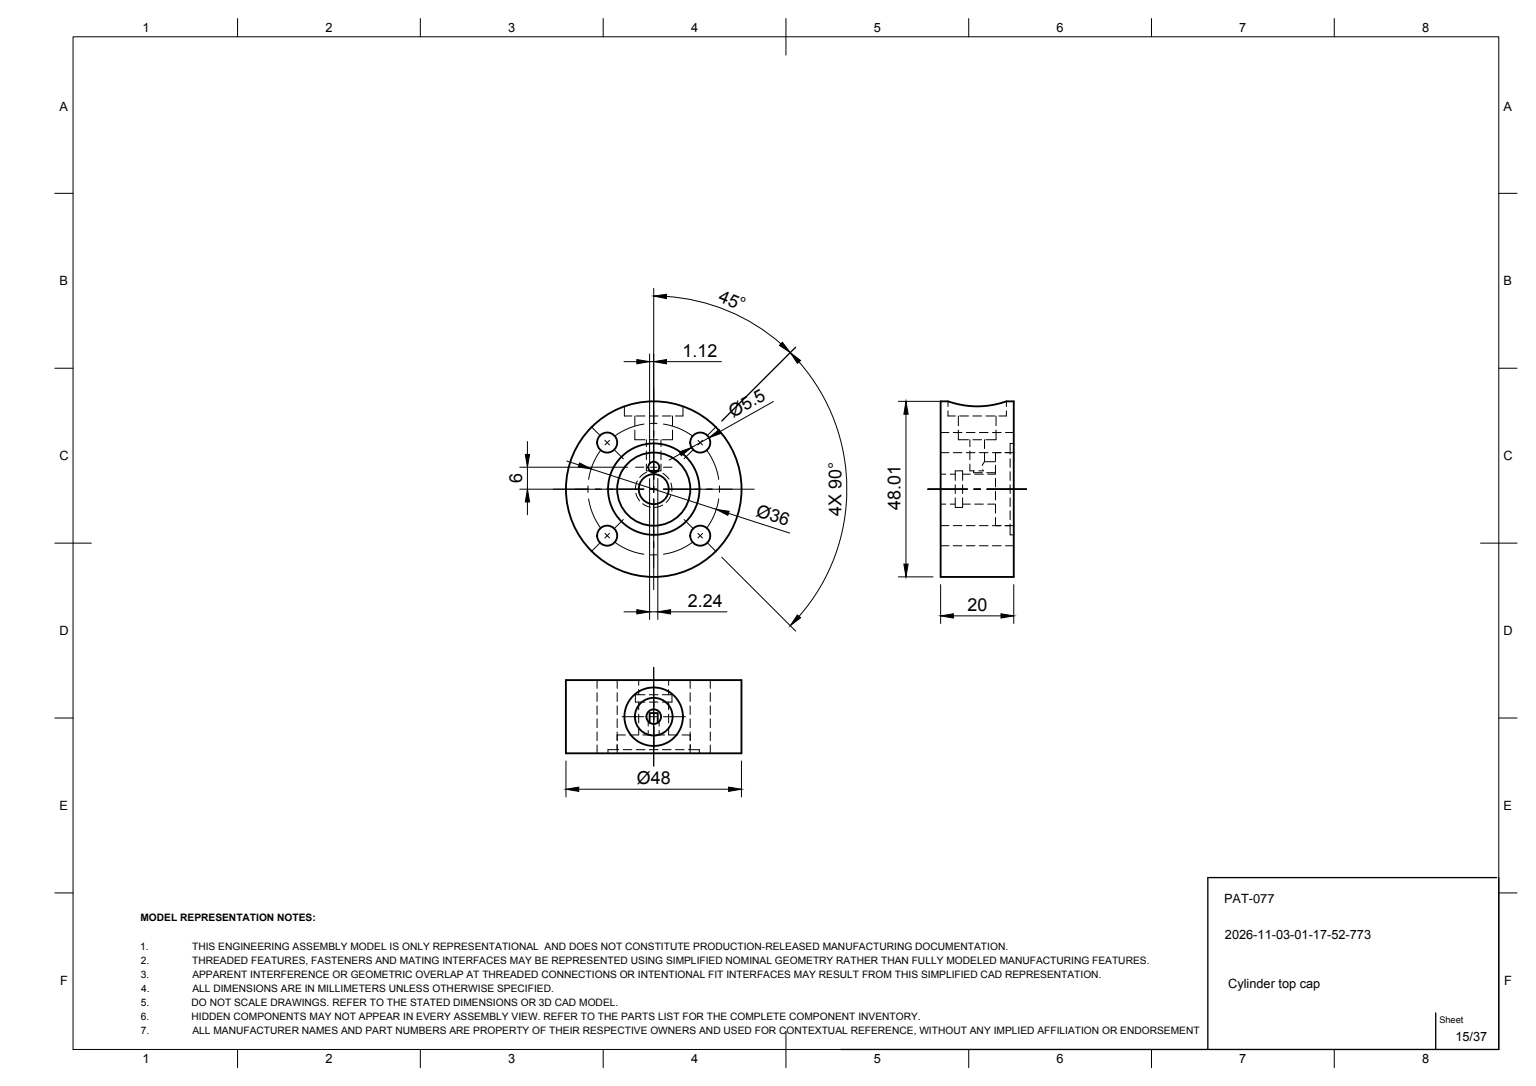
ISO-10303-21;
HEADER;
/* Generated by software containing ST-Developer
 * from STEP Tools, Inc. (www.steptools.com) 
 */

FILE_DESCRIPTION(
/* description */ ('Pallet stop with pneumatic fitting'),
/* implementation_level */ '2;1');

FILE_NAME(
/* name */ 'Cylinder top cap.step',
/* time_stamp */ '2026-10-27T10:51:41-07:00',
/* author */ (''),
/* organization */ (''),
/* preprocessor_version */ 'ST-DEVELOPER v20.2',
/* originating_system */ 'Autodesk Translation Framework v15.17.0.0',
/* authorisation */ '');

FILE_SCHEMA (('AUTOMOTIVE_DESIGN { 1 0 10303 214 3 1 1 }'));
ENDSEC;

DATA;
#10=MECHANICAL_DESIGN_GEOMETRIC_PRESENTATION_REPRESENTATION('',(#367),#10265);
#284=B_SPLINE_CURVE_WITH_KNOTS('',3,(#9117,#9118,#9119,#9120,#9121,#9122,
#9123,#9124),.UNSPECIFIED.,.F.,.F.,(4,2,2,4),(-0.590204267533974,-0.538821839180455,
-0.508604823357851,-0.478387807535247),.UNSPECIFIED.);
#285=B_SPLINE_CURVE_WITH_KNOTS('',3,(#9128,#9129,#9130,#9131,#9132,#9133,
#9134,#9135,#9136,#9137,#9138,#9139,#9140,#9141,#9142,#9143,#9144,#9145,
#9146,#9147,#9148,#9149,#9150,#9151,#9152,#9153,#9154,#9155,#9156),
 .UNSPECIFIED.,.F.,.F.,(4,2,2,2,2,2,2,2,2,2,3,2,2,4),(-0.478387807535247,
-0.448170791712642,-0.417953775890038,-0.357519744244829,-0.298356824006226,
-0.239193903767623,-0.180030983529021,-0.120868063290418,-0.0604340316452091,
-0.0302170158226045,1.11022302462516E-16,0.0302170158226046,0.0604340316452092,
0.111816459998729),.UNSPECIFIED.);
#286=B_SPLINE_CURVE_WITH_KNOTS('',3,(#9177,#9178,#9179,#9180,#9181,#9182,
#9183,#9184,#9185,#9186,#9187,#9188,#9189,#9190,#9191,#9192,#9193,#9194,
#9195,#9196,#9197,#9198,#9199,#9200,#9201,#9202,#9203,#9204,#9205,#9206,
#9207,#9208,#9209,#9210),.UNSPECIFIED.,.T.,.F.,(4,2,2,2,2,2,2,2,2,2,2,2,
2,2,2,2,4),(0.,0.303950544978949,0.607901089957899,0.911710662439542,1.21552023492119,
1.51932980740283,1.82313937988447,2.12708992486342,2.43104046984237,2.73499101482132,
3.03894155980027,3.34275113228191,3.64656070476356,3.9503702772452,4.25417984972684,
4.55813039470579,4.86208093968474),.UNSPECIFIED.);
#303=SHAPE_REPRESENTATION_RELATIONSHIP('SRR','None',#10416,#335);
#335=ADVANCED_BREP_SHAPE_REPRESENTATION('',(#399),#10240);
#367=STYLED_ITEM('',(#10648),#399);
#399=MANIFOLD_SOLID_BREP('Body1',#5055);
#480=FACE_BOUND('',#1227,.T.);
#481=FACE_BOUND('',#1230,.T.);
#482=FACE_BOUND('',#1233,.T.);
#483=FACE_BOUND('',#1235,.T.);
#484=FACE_BOUND('',#1240,.T.);
#485=FACE_BOUND('',#1243,.T.);
#486=FACE_BOUND('',#1244,.T.);
#487=FACE_BOUND('',#1250,.T.);
#488=FACE_BOUND('',#1252,.T.);
#489=FACE_BOUND('',#1253,.T.);
#490=FACE_BOUND('',#1254,.T.);
#491=FACE_BOUND('',#1255,.T.);
#492=FACE_BOUND('',#1256,.T.);
#493=FACE_BOUND('',#1258,.T.);
#494=FACE_BOUND('',#1259,.T.);
#495=FACE_BOUND('',#1260,.T.);
#496=FACE_BOUND('',#1261,.T.);
#497=FACE_BOUND('',#1262,.T.);
#608=PLANE('',#5648);
#609=PLANE('',#5652);
#610=PLANE('',#5660);
#611=PLANE('',#5663);
#612=PLANE('',#5667);
#613=PLANE('',#5669);
#614=PLANE('',#5678);
#615=PLANE('',#5682);
#616=PLANE('',#5698);
#617=PLANE('',#5699);
#846=FACE_OUTER_BOUND('',#1221,.T.);
#847=FACE_OUTER_BOUND('',#1222,.T.);
#848=FACE_OUTER_BOUND('',#1223,.T.);
#849=FACE_OUTER_BOUND('',#1224,.T.);
#850=FACE_OUTER_BOUND('',#1225,.T.);
#851=FACE_OUTER_BOUND('',#1226,.T.);
#852=FACE_OUTER_BOUND('',#1228,.T.);
#853=FACE_OUTER_BOUND('',#1229,.T.);
#854=FACE_OUTER_BOUND('',#1231,.T.);
#855=FACE_OUTER_BOUND('',#1232,.T.);
#856=FACE_OUTER_BOUND('',#1234,.T.);
#857=FACE_OUTER_BOUND('',#1236,.T.);
#858=FACE_OUTER_BOUND('',#1237,.T.);
#859=FACE_OUTER_BOUND('',#1238,.T.);
#860=FACE_OUTER_BOUND('',#1239,.T.);
#861=FACE_OUTER_BOUND('',#1241,.T.);
#862=FACE_OUTER_BOUND('',#1242,.T.);
#863=FACE_OUTER_BOUND('',#1245,.T.);
#864=FACE_OUTER_BOUND('',#1246,.T.);
#865=FACE_OUTER_BOUND('',#1247,.T.);
#866=FACE_OUTER_BOUND('',#1248,.T.);
#867=FACE_OUTER_BOUND('',#1249,.T.);
#868=FACE_OUTER_BOUND('',#1251,.T.);
#869=FACE_OUTER_BOUND('',#1257,.T.);
#1221=EDGE_LOOP('',(#3844,#3845));
#1222=EDGE_LOOP('',(#3846,#3847,#3848,#3849,#3850,#3851,#3852,#3853));
#1223=EDGE_LOOP('',(#3854,#3855,#3856,#3857,#3858));
#1224=EDGE_LOOP('',(#3859,#3860,#3861,#3862,#3863,#3864,#3865));
#1225=EDGE_LOOP('',(#3866,#3867,#3868,#3869));
#1226=EDGE_LOOP('',(#3870));
#1227=EDGE_LOOP('',(#3871));
#1228=EDGE_LOOP('',(#3872,#3873,#3874,#3875));
#1229=EDGE_LOOP('',(#3876));
#1230=EDGE_LOOP('',(#3877));
#1231=EDGE_LOOP('',(#3878,#3879,#3880,#3881));
#1232=EDGE_LOOP('',(#3882));
#1233=EDGE_LOOP('',(#3883));
#1234=EDGE_LOOP('',(#3884));
#1235=EDGE_LOOP('',(#3885));
#1236=EDGE_LOOP('',(#3886,#3887,#3888,#3889));
#1237=EDGE_LOOP('',(#3890,#3891,#3892,#3893));
#1238=EDGE_LOOP('',(#3894,#3895,#3896,#3897));
#1239=EDGE_LOOP('',(#3898));
#1240=EDGE_LOOP('',(#3899));
#1241=EDGE_LOOP('',(#3900,#3901,#3902,#3903));
#1242=EDGE_LOOP('',(#3904));
#1243=EDGE_LOOP('',(#3905));
#1244=EDGE_LOOP('',(#3906));
#1245=EDGE_LOOP('',(#3907,#3908,#3909,#3910));
#1246=EDGE_LOOP('',(#3911,#3912,#3913,#3914));
#1247=EDGE_LOOP('',(#3915,#3916,#3917,#3918));
#1248=EDGE_LOOP('',(#3919,#3920,#3921,#3922));
#1249=EDGE_LOOP('',(#3923,#3924,#3925,#3926));
#1250=EDGE_LOOP('',(#3927));
#1251=EDGE_LOOP('',(#3928));
#1252=EDGE_LOOP('',(#3929));
#1253=EDGE_LOOP('',(#3930));
#1254=EDGE_LOOP('',(#3931));
#1255=EDGE_LOOP('',(#3932));
#1256=EDGE_LOOP('',(#3933));
#1257=EDGE_LOOP('',(#3934));
#1258=EDGE_LOOP('',(#3935));
#1259=EDGE_LOOP('',(#3936));
#1260=EDGE_LOOP('',(#3937));
#1261=EDGE_LOOP('',(#3938));
#1262=EDGE_LOOP('',(#3939));
#1609=LINE('',#9109,#1944);
#1610=LINE('',#9115,#1945);
#1611=LINE('',#9125,#1946);
#1612=LINE('',#9127,#1947);
#1613=LINE('',#9163,#1948);
#1614=LINE('',#9169,#1949);
#1615=LINE('',#9176,#1950);
#1616=LINE('',#9216,#1951);
#1617=LINE('',#9227,#1952);
#1618=LINE('',#9230,#1953);
#1619=LINE('',#9236,#1954);
#1620=LINE('',#9243,#1955);
#1621=LINE('',#9250,#1956);
#1622=LINE('',#9256,#1957);
#1623=LINE('',#9262,#1958);
#1624=LINE('',#9268,#1959);
#1625=LINE('',#9274,#1960);
#1944=VECTOR('',#6642,1.);
#1945=VECTOR('',#6649,0.15);
#1946=VECTOR('',#6650,1.);
#1947=VECTOR('',#6651,1.);
#1948=VECTOR('',#6660,0.2);
#1949=VECTOR('',#6667,0.515);
#1950=VECTOR('',#6676,0.8);
#1951=VECTOR('',#6683,0.5);
#1952=VECTOR('',#6698,0.41);
#1953=VECTOR('',#6701,0.41);
#1954=VECTOR('',#6708,1.25);
#1955=VECTOR('',#6717,1.);
#1956=VECTOR('',#6726,0.275);
#1957=VECTOR('',#6733,0.275);
#1958=VECTOR('',#6740,0.275);
#1959=VECTOR('',#6747,0.275);
#1960=VECTOR('',#6754,2.4);
#2254=CIRCLE('',#5649,0.15);
#2255=CIRCLE('',#5651,0.15);
#2256=CIRCLE('',#5653,0.2);
#2257=CIRCLE('',#5654,0.2);
#2258=CIRCLE('',#5656,0.2);
#2259=CIRCLE('',#5658,0.515);
#2260=CIRCLE('',#5659,0.515);
#2261=CIRCLE('',#5662,0.8);
#2262=CIRCLE('',#5665,0.5);
#2263=CIRCLE('',#5666,0.5);
#2264=CIRCLE('',#5668,0.41);
#2265=CIRCLE('',#5670,0.41);
#2266=CIRCLE('',#5672,0.41);
#2267=CIRCLE('',#5674,0.41);
#2268=CIRCLE('',#5676,1.25);
#2269=CIRCLE('',#5677,1.25);
#2270=CIRCLE('',#5679,1.);
#2271=CIRCLE('',#5681,1.);
#2272=CIRCLE('',#5684,0.275);
#2273=CIRCLE('',#5685,0.275);
#2274=CIRCLE('',#5687,0.275);
#2275=CIRCLE('',#5688,0.275);
#2276=CIRCLE('',#5690,0.275);
#2277=CIRCLE('',#5691,0.275);
#2278=CIRCLE('',#5693,0.275);
#2279=CIRCLE('',#5694,0.275);
#2280=CIRCLE('',#5696,2.4);
#2281=CIRCLE('',#5697,2.4);
#2550=VERTEX_POINT('',#9107);
#2551=VERTEX_POINT('',#9108);
#2552=VERTEX_POINT('',#9112);
#2553=VERTEX_POINT('',#9114);
#2554=VERTEX_POINT('',#9116);
#2555=VERTEX_POINT('',#9126);
#2556=VERTEX_POINT('',#9158);
#2557=VERTEX_POINT('',#9162);
#2558=VERTEX_POINT('',#9166);
#2559=VERTEX_POINT('',#9168);
#2560=VERTEX_POINT('',#9173);
#2561=VERTEX_POINT('',#9175);
#2562=VERTEX_POINT('',#9213);
#2563=VERTEX_POINT('',#9215);
#2564=VERTEX_POINT('',#9219);
#2565=VERTEX_POINT('',#9222);
#2566=VERTEX_POINT('',#9225);
#2567=VERTEX_POINT('',#9229);
#2568=VERTEX_POINT('',#9233);
#2569=VERTEX_POINT('',#9235);
#2570=VERTEX_POINT('',#9239);
#2571=VERTEX_POINT('',#9242);
#2572=VERTEX_POINT('',#9247);
#2573=VERTEX_POINT('',#9249);
#2574=VERTEX_POINT('',#9253);
#2575=VERTEX_POINT('',#9255);
#2576=VERTEX_POINT('',#9259);
#2577=VERTEX_POINT('',#9261);
#2578=VERTEX_POINT('',#9265);
#2579=VERTEX_POINT('',#9267);
#2580=VERTEX_POINT('',#9271);
#2581=VERTEX_POINT('',#9273);
#3021=EDGE_CURVE('',#2550,#2551,#1609,.T.);
#3022=EDGE_CURVE('',#2551,#2550,#2254,.T.);
#3023=EDGE_CURVE('',#2552,#2552,#2255,.T.);
#3024=EDGE_CURVE('',#2552,#2553,#1610,.T.);
#3025=EDGE_CURVE('',#2554,#2553,#284,.T.);
#3026=EDGE_CURVE('',#2551,#2554,#1611,.T.);
#3027=EDGE_CURVE('',#2555,#2550,#1612,.T.);
#3028=EDGE_CURVE('',#2553,#2555,#285,.T.);
#3029=EDGE_CURVE('',#2554,#2556,#2256,.T.);
#3030=EDGE_CURVE('',#2556,#2555,#2257,.T.);
#3031=EDGE_CURVE('',#2556,#2557,#1613,.T.);
#3032=EDGE_CURVE('',#2557,#2557,#2258,.T.);
#3033=EDGE_CURVE('',#2558,#2558,#2259,.T.);
#3034=EDGE_CURVE('',#2558,#2559,#1614,.T.);
#3035=EDGE_CURVE('',#2559,#2559,#2260,.T.);
#3036=EDGE_CURVE('',#2560,#2560,#2261,.T.);
#3037=EDGE_CURVE('',#2560,#2561,#1615,.T.);
#3038=EDGE_CURVE('',#2561,#2561,#286,.T.);
#3039=EDGE_CURVE('',#2562,#2562,#2262,.T.);
#3040=EDGE_CURVE('',#2562,#2563,#1616,.T.);
#3041=EDGE_CURVE('',#2563,#2563,#2263,.T.);
#3042=EDGE_CURVE('',#2564,#2564,#2264,.T.);
#3043=EDGE_CURVE('',#2565,#2565,#2265,.T.);
#3044=EDGE_CURVE('',#2566,#2566,#2266,.T.);
#3045=EDGE_CURVE('',#2566,#2565,#1617,.T.);
#3046=EDGE_CURVE('',#2564,#2567,#1618,.T.);
#3047=EDGE_CURVE('',#2567,#2567,#2267,.T.);
#3048=EDGE_CURVE('',#2568,#2568,#2268,.T.);
#3049=EDGE_CURVE('',#2568,#2569,#1619,.T.);
#3050=EDGE_CURVE('',#2569,#2569,#2269,.T.);
#3051=EDGE_CURVE('',#2570,#2570,#2270,.T.);
#3052=EDGE_CURVE('',#2570,#2571,#1620,.T.);
#3053=EDGE_CURVE('',#2571,#2571,#2271,.T.);
#3054=EDGE_CURVE('',#2572,#2572,#2272,.T.);
#3055=EDGE_CURVE('',#2572,#2573,#1621,.T.);
#3056=EDGE_CURVE('',#2573,#2573,#2273,.T.);
#3057=EDGE_CURVE('',#2574,#2574,#2274,.T.);
#3058=EDGE_CURVE('',#2574,#2575,#1622,.T.);
#3059=EDGE_CURVE('',#2575,#2575,#2275,.T.);
#3060=EDGE_CURVE('',#2576,#2576,#2276,.T.);
#3061=EDGE_CURVE('',#2576,#2577,#1623,.T.);
#3062=EDGE_CURVE('',#2577,#2577,#2277,.T.);
#3063=EDGE_CURVE('',#2578,#2578,#2278,.T.);
#3064=EDGE_CURVE('',#2578,#2579,#1624,.T.);
#3065=EDGE_CURVE('',#2579,#2579,#2279,.T.);
#3066=EDGE_CURVE('',#2580,#2580,#2280,.T.);
#3067=EDGE_CURVE('',#2580,#2581,#1625,.T.);
#3068=EDGE_CURVE('',#2581,#2581,#2281,.T.);
#3844=ORIENTED_EDGE('',*,*,#3021,.F.);
#3845=ORIENTED_EDGE('',*,*,#3022,.F.);
#3846=ORIENTED_EDGE('',*,*,#3023,.F.);
#3847=ORIENTED_EDGE('',*,*,#3024,.T.);
#3848=ORIENTED_EDGE('',*,*,#3025,.F.);
#3849=ORIENTED_EDGE('',*,*,#3026,.F.);
#3850=ORIENTED_EDGE('',*,*,#3022,.T.);
#3851=ORIENTED_EDGE('',*,*,#3027,.F.);
#3852=ORIENTED_EDGE('',*,*,#3028,.F.);
#3853=ORIENTED_EDGE('',*,*,#3024,.F.);
#3854=ORIENTED_EDGE('',*,*,#3027,.T.);
#3855=ORIENTED_EDGE('',*,*,#3021,.T.);
#3856=ORIENTED_EDGE('',*,*,#3026,.T.);
#3857=ORIENTED_EDGE('',*,*,#3029,.T.);
#3858=ORIENTED_EDGE('',*,*,#3030,.T.);
#3859=ORIENTED_EDGE('',*,*,#3025,.T.);
#3860=ORIENTED_EDGE('',*,*,#3028,.T.);
#3861=ORIENTED_EDGE('',*,*,#3030,.F.);
#3862=ORIENTED_EDGE('',*,*,#3031,.T.);
#3863=ORIENTED_EDGE('',*,*,#3032,.F.);
#3864=ORIENTED_EDGE('',*,*,#3031,.F.);
#3865=ORIENTED_EDGE('',*,*,#3029,.F.);
#3866=ORIENTED_EDGE('',*,*,#3033,.F.);
#3867=ORIENTED_EDGE('',*,*,#3034,.T.);
#3868=ORIENTED_EDGE('',*,*,#3035,.F.);
#3869=ORIENTED_EDGE('',*,*,#3034,.F.);
#3870=ORIENTED_EDGE('',*,*,#3033,.T.);
#3871=ORIENTED_EDGE('',*,*,#3032,.T.);
#3872=ORIENTED_EDGE('',*,*,#3036,.F.);
#3873=ORIENTED_EDGE('',*,*,#3037,.T.);
#3874=ORIENTED_EDGE('',*,*,#3038,.F.);
#3875=ORIENTED_EDGE('',*,*,#3037,.F.);
#3876=ORIENTED_EDGE('',*,*,#3036,.T.);
#3877=ORIENTED_EDGE('',*,*,#3035,.T.);
#3878=ORIENTED_EDGE('',*,*,#3039,.F.);
#3879=ORIENTED_EDGE('',*,*,#3040,.T.);
#3880=ORIENTED_EDGE('',*,*,#3041,.T.);
#3881=ORIENTED_EDGE('',*,*,#3040,.F.);
#3882=ORIENTED_EDGE('',*,*,#3041,.F.);
#3883=ORIENTED_EDGE('',*,*,#3042,.F.);
#3884=ORIENTED_EDGE('',*,*,#3039,.T.);
#3885=ORIENTED_EDGE('',*,*,#3043,.F.);
#3886=ORIENTED_EDGE('',*,*,#3044,.F.);
#3887=ORIENTED_EDGE('',*,*,#3045,.T.);
#3888=ORIENTED_EDGE('',*,*,#3043,.T.);
#3889=ORIENTED_EDGE('',*,*,#3045,.F.);
#3890=ORIENTED_EDGE('',*,*,#3042,.T.);
#3891=ORIENTED_EDGE('',*,*,#3046,.T.);
#3892=ORIENTED_EDGE('',*,*,#3047,.F.);
#3893=ORIENTED_EDGE('',*,*,#3046,.F.);
#3894=ORIENTED_EDGE('',*,*,#3048,.F.);
#3895=ORIENTED_EDGE('',*,*,#3049,.T.);
#3896=ORIENTED_EDGE('',*,*,#3050,.T.);
#3897=ORIENTED_EDGE('',*,*,#3049,.F.);
#3898=ORIENTED_EDGE('',*,*,#3050,.F.);
#3899=ORIENTED_EDGE('',*,*,#3051,.F.);
#3900=ORIENTED_EDGE('',*,*,#3051,.T.);
#3901=ORIENTED_EDGE('',*,*,#3052,.T.);
#3902=ORIENTED_EDGE('',*,*,#3053,.T.);
#3903=ORIENTED_EDGE('',*,*,#3052,.F.);
#3904=ORIENTED_EDGE('',*,*,#3053,.F.);
#3905=ORIENTED_EDGE('',*,*,#3023,.T.);
#3906=ORIENTED_EDGE('',*,*,#3044,.T.);
#3907=ORIENTED_EDGE('',*,*,#3054,.F.);
#3908=ORIENTED_EDGE('',*,*,#3055,.T.);
#3909=ORIENTED_EDGE('',*,*,#3056,.F.);
#3910=ORIENTED_EDGE('',*,*,#3055,.F.);
#3911=ORIENTED_EDGE('',*,*,#3057,.F.);
#3912=ORIENTED_EDGE('',*,*,#3058,.T.);
#3913=ORIENTED_EDGE('',*,*,#3059,.F.);
#3914=ORIENTED_EDGE('',*,*,#3058,.F.);
#3915=ORIENTED_EDGE('',*,*,#3060,.F.);
#3916=ORIENTED_EDGE('',*,*,#3061,.T.);
#3917=ORIENTED_EDGE('',*,*,#3062,.F.);
#3918=ORIENTED_EDGE('',*,*,#3061,.F.);
#3919=ORIENTED_EDGE('',*,*,#3063,.F.);
#3920=ORIENTED_EDGE('',*,*,#3064,.T.);
#3921=ORIENTED_EDGE('',*,*,#3065,.F.);
#3922=ORIENTED_EDGE('',*,*,#3064,.F.);
#3923=ORIENTED_EDGE('',*,*,#3066,.F.);
#3924=ORIENTED_EDGE('',*,*,#3067,.T.);
#3925=ORIENTED_EDGE('',*,*,#3068,.T.);
#3926=ORIENTED_EDGE('',*,*,#3067,.F.);
#3927=ORIENTED_EDGE('',*,*,#3038,.T.);
#3928=ORIENTED_EDGE('',*,*,#3066,.T.);
#3929=ORIENTED_EDGE('',*,*,#3047,.T.);
#3930=ORIENTED_EDGE('',*,*,#3056,.T.);
#3931=ORIENTED_EDGE('',*,*,#3059,.T.);
#3932=ORIENTED_EDGE('',*,*,#3062,.T.);
#3933=ORIENTED_EDGE('',*,*,#3065,.T.);
#3934=ORIENTED_EDGE('',*,*,#3068,.F.);
#3935=ORIENTED_EDGE('',*,*,#3048,.T.);
#3936=ORIENTED_EDGE('',*,*,#3054,.T.);
#3937=ORIENTED_EDGE('',*,*,#3057,.T.);
#3938=ORIENTED_EDGE('',*,*,#3060,.T.);
#3939=ORIENTED_EDGE('',*,*,#3063,.T.);
#4668=CYLINDRICAL_SURFACE('',#5650,0.15);
#4669=CYLINDRICAL_SURFACE('',#5655,0.2);
#4670=CYLINDRICAL_SURFACE('',#5657,0.515);
#4671=CYLINDRICAL_SURFACE('',#5661,0.8);
#4672=CYLINDRICAL_SURFACE('',#5664,0.5);
#4673=CYLINDRICAL_SURFACE('',#5671,0.41);
#4674=CYLINDRICAL_SURFACE('',#5673,0.41);
#4675=CYLINDRICAL_SURFACE('',#5675,1.25);
#4676=CYLINDRICAL_SURFACE('',#5680,1.);
#4677=CYLINDRICAL_SURFACE('',#5683,0.275);
#4678=CYLINDRICAL_SURFACE('',#5686,0.275);
#4679=CYLINDRICAL_SURFACE('',#5689,0.275);
#4680=CYLINDRICAL_SURFACE('',#5692,0.275);
#4681=CYLINDRICAL_SURFACE('',#5695,2.4);
#4841=ADVANCED_FACE('',(#846),#608,.F.);
#4842=ADVANCED_FACE('',(#847),#4668,.F.);
#4843=ADVANCED_FACE('',(#848),#609,.T.);
#4844=ADVANCED_FACE('',(#849),#4669,.F.);
#4845=ADVANCED_FACE('',(#850),#4670,.F.);
#4846=ADVANCED_FACE('',(#851,#480),#610,.T.);
#4847=ADVANCED_FACE('',(#852),#4671,.F.);
#4848=ADVANCED_FACE('',(#853,#481),#611,.T.);
#4849=ADVANCED_FACE('',(#854),#4672,.F.);
#4850=ADVANCED_FACE('',(#855,#482),#612,.F.);
#4851=ADVANCED_FACE('',(#856,#483),#613,.T.);
#4852=ADVANCED_FACE('',(#857),#4673,.F.);
#4853=ADVANCED_FACE('',(#858),#4674,.F.);
#4854=ADVANCED_FACE('',(#859),#4675,.F.);
#4855=ADVANCED_FACE('',(#860,#484),#614,.F.);
#4856=ADVANCED_FACE('',(#861),#4676,.F.);
#4857=ADVANCED_FACE('',(#862,#485,#486),#615,.F.);
#4858=ADVANCED_FACE('',(#863),#4677,.F.);
#4859=ADVANCED_FACE('',(#864),#4678,.F.);
#4860=ADVANCED_FACE('',(#865),#4679,.F.);
#4861=ADVANCED_FACE('',(#866),#4680,.F.);
#4862=ADVANCED_FACE('',(#867,#487),#4681,.T.);
#4863=ADVANCED_FACE('',(#868,#488,#489,#490,#491,#492),#616,.T.);
#4864=ADVANCED_FACE('',(#869,#493,#494,#495,#496,#497),#617,.F.);
#5055=CLOSED_SHELL('',(#4841,#4842,#4843,#4844,#4845,#4846,#4847,#4848,
#4849,#4850,#4851,#4852,#4853,#4854,#4855,#4856,#4857,#4858,#4859,#4860,
#4861,#4862,#4863,#4864));
#5647=AXIS2_PLACEMENT_3D('',#9105,#6638,#6639);
#5648=AXIS2_PLACEMENT_3D('',#9106,#6640,#6641);
#5649=AXIS2_PLACEMENT_3D('',#9110,#6643,#6644);
#5650=AXIS2_PLACEMENT_3D('',#9111,#6645,#6646);
#5651=AXIS2_PLACEMENT_3D('',#9113,#6647,#6648);
#5652=AXIS2_PLACEMENT_3D('',#9157,#6652,#6653);
#5653=AXIS2_PLACEMENT_3D('',#9159,#6654,#6655);
#5654=AXIS2_PLACEMENT_3D('',#9160,#6656,#6657);
#5655=AXIS2_PLACEMENT_3D('',#9161,#6658,#6659);
#5656=AXIS2_PLACEMENT_3D('',#9164,#6661,#6662);
#5657=AXIS2_PLACEMENT_3D('',#9165,#6663,#6664);
#5658=AXIS2_PLACEMENT_3D('',#9167,#6665,#6666);
#5659=AXIS2_PLACEMENT_3D('',#9170,#6668,#6669);
#5660=AXIS2_PLACEMENT_3D('',#9171,#6670,#6671);
#5661=AXIS2_PLACEMENT_3D('',#9172,#6672,#6673);
#5662=AXIS2_PLACEMENT_3D('',#9174,#6674,#6675);
#5663=AXIS2_PLACEMENT_3D('',#9211,#6677,#6678);
#5664=AXIS2_PLACEMENT_3D('',#9212,#6679,#6680);
#5665=AXIS2_PLACEMENT_3D('',#9214,#6681,#6682);
#5666=AXIS2_PLACEMENT_3D('',#9217,#6684,#6685);
#5667=AXIS2_PLACEMENT_3D('',#9218,#6686,#6687);
#5668=AXIS2_PLACEMENT_3D('',#9220,#6688,#6689);
#5669=AXIS2_PLACEMENT_3D('',#9221,#6690,#6691);
#5670=AXIS2_PLACEMENT_3D('',#9223,#6692,#6693);
#5671=AXIS2_PLACEMENT_3D('',#9224,#6694,#6695);
#5672=AXIS2_PLACEMENT_3D('',#9226,#6696,#6697);
#5673=AXIS2_PLACEMENT_3D('',#9228,#6699,#6700);
#5674=AXIS2_PLACEMENT_3D('',#9231,#6702,#6703);
#5675=AXIS2_PLACEMENT_3D('',#9232,#6704,#6705);
#5676=AXIS2_PLACEMENT_3D('',#9234,#6706,#6707);
#5677=AXIS2_PLACEMENT_3D('',#9237,#6709,#6710);
#5678=AXIS2_PLACEMENT_3D('',#9238,#6711,#6712);
#5679=AXIS2_PLACEMENT_3D('',#9240,#6713,#6714);
#5680=AXIS2_PLACEMENT_3D('',#9241,#6715,#6716);
#5681=AXIS2_PLACEMENT_3D('',#9244,#6718,#6719);
#5682=AXIS2_PLACEMENT_3D('',#9245,#6720,#6721);
#5683=AXIS2_PLACEMENT_3D('',#9246,#6722,#6723);
#5684=AXIS2_PLACEMENT_3D('',#9248,#6724,#6725);
#5685=AXIS2_PLACEMENT_3D('',#9251,#6727,#6728);
#5686=AXIS2_PLACEMENT_3D('',#9252,#6729,#6730);
#5687=AXIS2_PLACEMENT_3D('',#9254,#6731,#6732);
#5688=AXIS2_PLACEMENT_3D('',#9257,#6734,#6735);
#5689=AXIS2_PLACEMENT_3D('',#9258,#6736,#6737);
#5690=AXIS2_PLACEMENT_3D('',#9260,#6738,#6739);
#5691=AXIS2_PLACEMENT_3D('',#9263,#6741,#6742);
#5692=AXIS2_PLACEMENT_3D('',#9264,#6743,#6744);
#5693=AXIS2_PLACEMENT_3D('',#9266,#6745,#6746);
#5694=AXIS2_PLACEMENT_3D('',#9269,#6748,#6749);
#5695=AXIS2_PLACEMENT_3D('',#9270,#6750,#6751);
#5696=AXIS2_PLACEMENT_3D('',#9272,#6752,#6753);
#5697=AXIS2_PLACEMENT_3D('',#9275,#6755,#6756);
#5698=AXIS2_PLACEMENT_3D('',#9276,#6757,#6758);
#5699=AXIS2_PLACEMENT_3D('',#9277,#6759,#6760);
#6638=DIRECTION('axis',(0.,0.,1.));
#6639=DIRECTION('refdir',(1.,0.,0.));
#6640=DIRECTION('center_axis',(0.,0.,1.));
#6641=DIRECTION('ref_axis',(1.,0.,0.));
#6642=DIRECTION('',(-1.,0.,0.));
#6643=DIRECTION('center_axis',(0.,0.,1.));
#6644=DIRECTION('ref_axis',(1.,0.,0.));
#6645=DIRECTION('center_axis',(0.,0.,1.));
#6646=DIRECTION('ref_axis',(1.,0.,0.));
#6647=DIRECTION('center_axis',(0.,0.,1.));
#6648=DIRECTION('ref_axis',(1.,0.,0.));
#6649=DIRECTION('',(0.,0.,1.));
#6650=DIRECTION('',(0.,0.,-1.));
#6651=DIRECTION('',(0.,0.,1.));
#6652=DIRECTION('center_axis',(0.,1.,0.));
#6653=DIRECTION('ref_axis',(1.,0.,0.));
#6654=DIRECTION('center_axis',(0.,1.,0.));
#6655=DIRECTION('ref_axis',(1.,0.,0.));
#6656=DIRECTION('center_axis',(0.,1.,0.));
#6657=DIRECTION('ref_axis',(1.,0.,0.));
#6658=DIRECTION('center_axis',(0.,1.,0.));
#6659=DIRECTION('ref_axis',(1.,0.,0.));
#6660=DIRECTION('',(0.,1.,0.));
#6661=DIRECTION('center_axis',(0.,-1.,0.));
#6662=DIRECTION('ref_axis',(1.,0.,0.));
#6663=DIRECTION('center_axis',(0.,1.,0.));
#6664=DIRECTION('ref_axis',(1.,0.,0.));
#6665=DIRECTION('center_axis',(0.,1.,0.));
#6666=DIRECTION('ref_axis',(1.,0.,0.));
#6667=DIRECTION('',(0.,1.,0.));
#6668=DIRECTION('center_axis',(0.,-1.,0.));
#6669=DIRECTION('ref_axis',(1.,0.,0.));
#6670=DIRECTION('center_axis',(0.,1.,0.));
#6671=DIRECTION('ref_axis',(1.,0.,0.));
#6672=DIRECTION('center_axis',(0.,1.,0.));
#6673=DIRECTION('ref_axis',(1.,0.,0.));
#6674=DIRECTION('center_axis',(0.,1.,0.));
#6675=DIRECTION('ref_axis',(1.,0.,0.));
#6676=DIRECTION('',(0.,1.,0.));
#6677=DIRECTION('center_axis',(0.,1.,0.));
#6678=DIRECTION('ref_axis',(1.,0.,0.));
#6679=DIRECTION('center_axis',(0.,0.,1.));
#6680=DIRECTION('ref_axis',(1.,0.,0.));
#6681=DIRECTION('center_axis',(0.,0.,1.));
#6682=DIRECTION('ref_axis',(1.,0.,0.));
#6683=DIRECTION('',(0.,0.,1.));
#6684=DIRECTION('center_axis',(0.,0.,1.));
#6685=DIRECTION('ref_axis',(1.,0.,0.));
#6686=DIRECTION('center_axis',(0.,0.,1.));
#6687=DIRECTION('ref_axis',(1.,0.,0.));
#6688=DIRECTION('center_axis',(0.,0.,-1.));
#6689=DIRECTION('ref_axis',(1.,0.,0.));
#6690=DIRECTION('center_axis',(0.,0.,1.));
#6691=DIRECTION('ref_axis',(1.,0.,0.));
#6692=DIRECTION('center_axis',(0.,0.,1.));
#6693=DIRECTION('ref_axis',(1.,0.,0.));
#6694=DIRECTION('center_axis',(0.,0.,1.));
#6695=DIRECTION('ref_axis',(1.,0.,0.));
#6696=DIRECTION('center_axis',(0.,0.,1.));
#6697=DIRECTION('ref_axis',(1.,0.,0.));
#6698=DIRECTION('',(0.,0.,1.));
#6699=DIRECTION('center_axis',(0.,0.,1.));
#6700=DIRECTION('ref_axis',(1.,0.,0.));
#6701=DIRECTION('',(0.,0.,1.));
#6702=DIRECTION('center_axis',(0.,0.,-1.));
#6703=DIRECTION('ref_axis',(1.,0.,0.));
#6704=DIRECTION('center_axis',(0.,0.,1.));
#6705=DIRECTION('ref_axis',(1.,0.,0.));
#6706=DIRECTION('center_axis',(0.,0.,1.));
#6707=DIRECTION('ref_axis',(1.,0.,0.));
#6708=DIRECTION('',(0.,0.,1.));
#6709=DIRECTION('center_axis',(0.,0.,1.));
#6710=DIRECTION('ref_axis',(1.,0.,0.));
#6711=DIRECTION('center_axis',(0.,0.,1.));
#6712=DIRECTION('ref_axis',(1.,0.,0.));
#6713=DIRECTION('center_axis',(0.,0.,-1.));
#6714=DIRECTION('ref_axis',(1.,0.,0.));
#6715=DIRECTION('center_axis',(0.,0.,1.));
#6716=DIRECTION('ref_axis',(1.,0.,0.));
#6717=DIRECTION('',(0.,0.,1.));
#6718=DIRECTION('center_axis',(0.,0.,1.));
#6719=DIRECTION('ref_axis',(1.,0.,0.));
#6720=DIRECTION('center_axis',(0.,0.,1.));
#6721=DIRECTION('ref_axis',(1.,0.,0.));
#6722=DIRECTION('center_axis',(0.,0.,1.));
#6723=DIRECTION('ref_axis',(1.,0.,0.));
#6724=DIRECTION('center_axis',(0.,0.,1.));
#6725=DIRECTION('ref_axis',(1.,0.,0.));
#6726=DIRECTION('',(0.,0.,1.));
#6727=DIRECTION('center_axis',(0.,0.,-1.));
#6728=DIRECTION('ref_axis',(1.,0.,0.));
#6729=DIRECTION('center_axis',(0.,0.,1.));
#6730=DIRECTION('ref_axis',(1.,0.,0.));
#6731=DIRECTION('center_axis',(0.,0.,1.));
#6732=DIRECTION('ref_axis',(1.,0.,0.));
#6733=DIRECTION('',(0.,0.,1.));
#6734=DIRECTION('center_axis',(0.,0.,-1.));
#6735=DIRECTION('ref_axis',(1.,0.,0.));
#6736=DIRECTION('center_axis',(0.,0.,1.));
#6737=DIRECTION('ref_axis',(1.,0.,0.));
#6738=DIRECTION('center_axis',(0.,0.,1.));
#6739=DIRECTION('ref_axis',(1.,0.,0.));
#6740=DIRECTION('',(0.,0.,1.));
#6741=DIRECTION('center_axis',(0.,0.,-1.));
#6742=DIRECTION('ref_axis',(1.,0.,0.));
#6743=DIRECTION('center_axis',(0.,0.,1.));
#6744=DIRECTION('ref_axis',(1.,0.,0.));
#6745=DIRECTION('center_axis',(0.,0.,1.));
#6746=DIRECTION('ref_axis',(1.,0.,0.));
#6747=DIRECTION('',(0.,0.,1.));
#6748=DIRECTION('center_axis',(0.,0.,-1.));
#6749=DIRECTION('ref_axis',(1.,0.,0.));
#6750=DIRECTION('center_axis',(0.,0.,1.));
#6751=DIRECTION('ref_axis',(1.,0.,0.));
#6752=DIRECTION('center_axis',(0.,0.,1.));
#6753=DIRECTION('ref_axis',(1.,0.,0.));
#6754=DIRECTION('',(0.,0.,-1.));
#6755=DIRECTION('center_axis',(0.,0.,1.));
#6756=DIRECTION('ref_axis',(1.,0.,0.));
#6757=DIRECTION('center_axis',(0.,0.,1.));
#6758=DIRECTION('ref_axis',(1.,0.,0.));
#6759=DIRECTION('center_axis',(0.,0.,1.));
#6760=DIRECTION('ref_axis',(1.,0.,0.));
#9105=CARTESIAN_POINT('',(0.,0.,0.));
#9106=CARTESIAN_POINT('Origin',(4.,4.6,9.1));
#9107=CARTESIAN_POINT('',(4.11180339887499,4.5,9.1));
#9108=CARTESIAN_POINT('',(3.88819660112501,4.5,9.1));
#9109=CARTESIAN_POINT('',(4.,4.5,9.1));
#9110=CARTESIAN_POINT('Origin',(4.,4.6,9.1));
#9111=CARTESIAN_POINT('Origin',(4.,4.6,8.4));
#9112=CARTESIAN_POINT('',(3.85,4.6,8.5));
#9113=CARTESIAN_POINT('Origin',(4.,4.6,8.5));
#9114=CARTESIAN_POINT('',(3.85,4.6,8.86771243444677));
#9115=CARTESIAN_POINT('',(3.85,4.6,8.4));
#9116=CARTESIAN_POINT('',(3.88819660112501,4.5,8.83416876048223));
#9117=CARTESIAN_POINT('Ctrl Pts',(3.88819660112501,4.5,8.83416876048223));
#9118=CARTESIAN_POINT('Ctrl Pts',(3.87757657209989,4.5118735534116,8.84132878259032));
#9119=CARTESIAN_POINT('Ctrl Pts',(3.86846014424429,4.52597563413084,8.84907123479525));
#9120=CARTESIAN_POINT('Ctrl Pts',(3.85804355837321,4.55054285102637,8.85901486480765));
#9121=CARTESIAN_POINT('Ctrl Pts',(3.8550467625566,4.56012752110791,8.86217045472001));
#9122=CARTESIAN_POINT('Ctrl Pts',(3.85102541664982,4.57981886189345,8.86652445682054));
#9123=CARTESIAN_POINT('Ctrl Pts',(3.85,4.58992766139246,8.86771243444677));
#9124=CARTESIAN_POINT('Ctrl Pts',(3.85,4.6,8.86771243444677));
#9125=CARTESIAN_POINT('',(3.88819660112501,4.5,8.4));
#9126=CARTESIAN_POINT('',(4.11180339887499,4.5,8.83416876048223));
#9127=CARTESIAN_POINT('',(4.11180339887499,4.5,8.4));
#9128=CARTESIAN_POINT('Ctrl Pts',(3.85,4.6,8.86771243444677));
#9129=CARTESIAN_POINT('Ctrl Pts',(3.85,4.61007233860753,8.86771243444677));
#9130=CARTESIAN_POINT('Ctrl Pts',(3.85102541664981,4.62018113810654,8.86652445682054));
#9131=CARTESIAN_POINT('Ctrl Pts',(3.85504676255659,4.63987247889209,8.86217045472001));
#9132=CARTESIAN_POINT('Ctrl Pts',(3.85804355837321,4.64945714897362,8.85901486480765));
#9133=CARTESIAN_POINT('Ctrl Pts',(3.8696156276414,4.67674954008529,8.84796821509873));
#9134=CARTESIAN_POINT('Ctrl Pts',(3.88090702862397,4.69303906297994,8.83859067358653));
#9135=CARTESIAN_POINT('Ctrl Pts',(3.90668694057098,4.71881897492694,8.82246422388431));
#9136=CARTESIAN_POINT('Ctrl Pts',(3.9230088222236,4.73027430044143,8.81441378257927));
#9137=CARTESIAN_POINT('Ctrl Pts',(3.95978537347009,4.74588290014714,8.80314301976006));
#9138=CARTESIAN_POINT('Ctrl Pts',(3.98027902658713,4.75,8.8));
#9139=CARTESIAN_POINT('Ctrl Pts',(4.01972097341287,4.75,8.8));
#9140=CARTESIAN_POINT('Ctrl Pts',(4.04021462652991,4.74588290014714,8.80314301976006));
#9141=CARTESIAN_POINT('Ctrl Pts',(4.0769911777764,4.73027430044143,8.81441378257927));
#9142=CARTESIAN_POINT('Ctrl Pts',(4.09331305942902,4.71881897492694,8.82246422388431));
#9143=CARTESIAN_POINT('Ctrl Pts',(4.11909297137603,4.69303906297994,8.83859067358653));
#9144=CARTESIAN_POINT('Ctrl Pts',(4.1303843723586,4.67674954008529,8.84796821509873));
#9145=CARTESIAN_POINT('Ctrl Pts',(4.14195644162679,4.64945714897363,8.85901486480765));
#9146=CARTESIAN_POINT('Ctrl Pts',(4.1449532374434,4.63987247889209,8.86217045472001));
#9147=CARTESIAN_POINT('Ctrl Pts',(4.14897458335018,4.62018113810655,8.86652445682054));
#9148=CARTESIAN_POINT('Ctrl Pts',(4.15,4.61007233860753,8.86771243444677));
#9149=CARTESIAN_POINT('Ctrl Pts',(4.15,4.6,8.86771243444677));
#9150=CARTESIAN_POINT('Ctrl Pts',(4.15,4.58992766139246,8.86771243444677));
#9151=CARTESIAN_POINT('Ctrl Pts',(4.14897458335018,4.57981886189345,8.86652445682054));
#9152=CARTESIAN_POINT('Ctrl Pts',(4.1449532374434,4.56012752110791,8.86217045472001));
#9153=CARTESIAN_POINT('Ctrl Pts',(4.14195644162679,4.55054285102637,8.85901486480765));
#9154=CARTESIAN_POINT('Ctrl Pts',(4.13153985575571,4.52597563413084,8.84907123479525));
#9155=CARTESIAN_POINT('Ctrl Pts',(4.12242342790011,4.5118735534116,8.84132878259032));
#9156=CARTESIAN_POINT('Ctrl Pts',(4.11180339887499,4.5,8.83416876048223));
#9157=CARTESIAN_POINT('Origin',(4.,4.5,9.));
#9158=CARTESIAN_POINT('',(3.8,4.5,9.));
#9159=CARTESIAN_POINT('Origin',(4.,4.5,9.));
#9160=CARTESIAN_POINT('Origin',(4.,4.5,9.));
#9161=CARTESIAN_POINT('Origin',(4.,4.5,9.));
#9162=CARTESIAN_POINT('',(3.8,5.35,9.));
#9163=CARTESIAN_POINT('',(3.8,4.5,9.));
#9164=CARTESIAN_POINT('Origin',(4.,5.35,9.));
#9165=CARTESIAN_POINT('Origin',(4.,5.35,9.));
#9166=CARTESIAN_POINT('',(3.485,5.35,9.));
#9167=CARTESIAN_POINT('Origin',(4.,5.35,9.));
#9168=CARTESIAN_POINT('',(3.485,6.,9.));
#9169=CARTESIAN_POINT('',(3.485,5.35,9.));
#9170=CARTESIAN_POINT('Origin',(4.,6.,9.));
#9171=CARTESIAN_POINT('Origin',(4.,5.35,9.));
#9172=CARTESIAN_POINT('Origin',(4.,6.,9.));
#9173=CARTESIAN_POINT('',(3.2,6.,9.));
#9174=CARTESIAN_POINT('Origin',(4.,6.,9.));
#9175=CARTESIAN_POINT('',(3.2,6.26274169979695,9.));
#9176=CARTESIAN_POINT('',(3.2,6.,9.));
#9177=CARTESIAN_POINT('Ctrl Pts',(3.2,6.26274169979695,9.));
#9178=CARTESIAN_POINT('Ctrl Pts',(3.2,6.26274169979695,8.89868315167368));
#9179=CARTESIAN_POINT('Ctrl Pts',(3.22040772858495,6.270261426297,8.79119842122918));
#9180=CARTESIAN_POINT('Ctrl Pts',(3.30227767389892,6.29674433020986,8.59435745603384));
#9181=CARTESIAN_POINT('Ctrl Pts',(3.36370361600024,6.31525508485039,8.50492553410129));
#9182=CARTESIAN_POINT('Ctrl Pts',(3.50489278468399,6.34949848812546,8.36373636541753));
#9183=CARTESIAN_POINT('Ctrl Pts',(3.59433775043408,6.36754956424272,8.30228521110673));
#9184=CARTESIAN_POINT('Ctrl Pts',(3.79122709022331,6.39296190354765,8.22039646335756));
#9185=CARTESIAN_POINT('Ctrl Pts',(3.89873014250612,6.4,8.2));
#9186=CARTESIAN_POINT('Ctrl Pts',(4.10126985749388,6.4,8.2));
#9187=CARTESIAN_POINT('Ctrl Pts',(4.20877290977668,6.39296190354765,8.22039646335756));
#9188=CARTESIAN_POINT('Ctrl Pts',(4.40566224956592,6.36754956424272,8.30228521110673));
#9189=CARTESIAN_POINT('Ctrl Pts',(4.49510721531601,6.34949848812546,8.36373636541753));
#9190=CARTESIAN_POINT('Ctrl Pts',(4.63629638399976,6.31525508485039,8.50492553410129));
#9191=CARTESIAN_POINT('Ctrl Pts',(4.69772232610108,6.29674433020987,8.59435745603384));
#9192=CARTESIAN_POINT('Ctrl Pts',(4.77959227141505,6.270261426297,8.79119842122918));
#9193=CARTESIAN_POINT('Ctrl Pts',(4.8,6.26274169979695,8.89868315167368));
#9194=CARTESIAN_POINT('Ctrl Pts',(4.8,6.26274169979695,9.10131684832632));
#9195=CARTESIAN_POINT('Ctrl Pts',(4.77959227141505,6.270261426297,9.20880157877082));
#9196=CARTESIAN_POINT('Ctrl Pts',(4.69772232610108,6.29674433020986,9.40564254396616));
#9197=CARTESIAN_POINT('Ctrl Pts',(4.63629638399976,6.31525508485039,9.49507446589871));
#9198=CARTESIAN_POINT('Ctrl Pts',(4.49510721531601,6.34949848812546,9.63626363458247));
#9199=CARTESIAN_POINT('Ctrl Pts',(4.40566224956592,6.36754956424272,9.69771478889327));
#9200=CARTESIAN_POINT('Ctrl Pts',(4.20877290977668,6.39296190354765,9.77960353664244));
#9201=CARTESIAN_POINT('Ctrl Pts',(4.10126985749388,6.4,9.8));
#9202=CARTESIAN_POINT('Ctrl Pts',(3.89873014250612,6.4,9.8));
#9203=CARTESIAN_POINT('Ctrl Pts',(3.79122709022331,6.39296190354765,9.77960353664244));
#9204=CARTESIAN_POINT('Ctrl Pts',(3.59433775043408,6.36754956424272,9.69771478889327));
#9205=CARTESIAN_POINT('Ctrl Pts',(3.50489278468399,6.34949848812546,9.63626363458247));
#9206=CARTESIAN_POINT('Ctrl Pts',(3.36370361600024,6.31525508485039,9.49507446589871));
#9207=CARTESIAN_POINT('Ctrl Pts',(3.30227767389892,6.29674433020986,9.40564254396616));
#9208=CARTESIAN_POINT('Ctrl Pts',(3.22040772858495,6.270261426297,9.20880157877082));
#9209=CARTESIAN_POINT('Ctrl Pts',(3.2,6.26274169979695,9.10131684832632));
#9210=CARTESIAN_POINT('Ctrl Pts',(3.2,6.26274169979695,9.));
#9211=CARTESIAN_POINT('Origin',(4.,6.,9.));
#9212=CARTESIAN_POINT('Origin',(4.,4.,9.4));
#9213=CARTESIAN_POINT('',(3.5,4.,9.4));
#9214=CARTESIAN_POINT('Origin',(4.,4.,9.4));
#9215=CARTESIAN_POINT('',(3.5,4.,9.6));
#9216=CARTESIAN_POINT('',(3.5,4.,9.4));
#9217=CARTESIAN_POINT('Origin',(4.,4.,9.6));
#9218=CARTESIAN_POINT('Origin',(4.,4.,9.6));
#9219=CARTESIAN_POINT('',(3.59,4.,9.6));
#9220=CARTESIAN_POINT('Origin',(4.,4.,9.6));
#9221=CARTESIAN_POINT('Origin',(4.,4.,9.4));
#9222=CARTESIAN_POINT('',(3.59,4.,9.4));
#9223=CARTESIAN_POINT('Origin',(4.,4.,9.4));
#9224=CARTESIAN_POINT('Origin',(4.,4.,8.4));
#9225=CARTESIAN_POINT('',(3.59,4.,8.5));
#9226=CARTESIAN_POINT('Origin',(4.,4.,8.5));
#9227=CARTESIAN_POINT('',(3.59,4.,8.4));
#9228=CARTESIAN_POINT('Origin',(4.,4.,8.4));
#9229=CARTESIAN_POINT('',(3.59,4.,10.));
#9230=CARTESIAN_POINT('',(3.59,4.,8.4));
#9231=CARTESIAN_POINT('Origin',(4.,4.,10.));
#9232=CARTESIAN_POINT('Origin',(4.,4.,8.));
#9233=CARTESIAN_POINT('',(2.75,4.,8.));
#9234=CARTESIAN_POINT('Origin',(4.,4.,8.));
#9235=CARTESIAN_POINT('',(2.75,4.,8.1));
#9236=CARTESIAN_POINT('',(2.75,4.,8.));
#9237=CARTESIAN_POINT('Origin',(4.,4.,8.1));
#9238=CARTESIAN_POINT('Origin',(4.,4.,8.1));
#9239=CARTESIAN_POINT('',(3.,4.,8.1));
#9240=CARTESIAN_POINT('Origin',(4.,4.,8.1));
#9241=CARTESIAN_POINT('Origin',(4.,4.,7.9));
#9242=CARTESIAN_POINT('',(3.,4.,8.5));
#9243=CARTESIAN_POINT('',(3.,4.,7.9));
#9244=CARTESIAN_POINT('Origin',(4.,4.,8.5));
#9245=CARTESIAN_POINT('Origin',(4.,4.,8.5));
#9246=CARTESIAN_POINT('Origin',(2.72720779386421,2.72720779386421,7.9));
#9247=CARTESIAN_POINT('',(2.45220779386421,2.72720779386421,8.));
#9248=CARTESIAN_POINT('Origin',(2.72720779386421,2.72720779386421,8.));
#9249=CARTESIAN_POINT('',(2.45220779386421,2.72720779386421,10.));
#9250=CARTESIAN_POINT('',(2.45220779386421,2.72720779386421,7.9));
#9251=CARTESIAN_POINT('Origin',(2.72720779386421,2.72720779386421,10.));
#9252=CARTESIAN_POINT('Origin',(2.72720779386421,5.27279220613579,7.9));
#9253=CARTESIAN_POINT('',(2.45220779386421,5.27279220613579,8.));
#9254=CARTESIAN_POINT('Origin',(2.72720779386421,5.27279220613579,8.));
#9255=CARTESIAN_POINT('',(2.45220779386421,5.27279220613579,10.));
#9256=CARTESIAN_POINT('',(2.45220779386421,5.27279220613579,7.9));
#9257=CARTESIAN_POINT('Origin',(2.72720779386421,5.27279220613579,10.));
#9258=CARTESIAN_POINT('Origin',(5.27279220613579,5.27279220613579,7.9));
#9259=CARTESIAN_POINT('',(4.99779220613579,5.27279220613579,8.));
#9260=CARTESIAN_POINT('Origin',(5.27279220613579,5.27279220613579,8.));
#9261=CARTESIAN_POINT('',(4.99779220613579,5.27279220613579,10.));
#9262=CARTESIAN_POINT('',(4.99779220613579,5.27279220613579,7.9));
#9263=CARTESIAN_POINT('Origin',(5.27279220613579,5.27279220613579,10.));
#9264=CARTESIAN_POINT('Origin',(5.27279220613578,2.72720779386421,7.9));
#9265=CARTESIAN_POINT('',(4.99779220613578,2.72720779386421,8.));
#9266=CARTESIAN_POINT('Origin',(5.27279220613578,2.72720779386421,8.));
#9267=CARTESIAN_POINT('',(4.99779220613578,2.72720779386421,10.));
#9268=CARTESIAN_POINT('',(4.99779220613578,2.72720779386421,7.9));
#9269=CARTESIAN_POINT('Origin',(5.27279220613578,2.72720779386421,10.));
#9270=CARTESIAN_POINT('Origin',(4.,4.,8.));
#9271=CARTESIAN_POINT('',(1.6,4.,10.));
#9272=CARTESIAN_POINT('Origin',(4.,4.,10.));
#9273=CARTESIAN_POINT('',(1.6,4.,8.));
#9274=CARTESIAN_POINT('',(1.6,4.,8.));
#9275=CARTESIAN_POINT('Origin',(4.,4.,8.));
#9276=CARTESIAN_POINT('Origin',(4.,4.,10.));
#9277=CARTESIAN_POINT('Origin',(4.,4.,8.));
#10202=UNCERTAINTY_MEASURE_WITH_UNIT(LENGTH_MEASURE(0.001),#10266,
'DISTANCE_ACCURACY_VALUE',
'Maximum model space distance between geometric entities at asserted c
onnectivities');
#10227=UNCERTAINTY_MEASURE_WITH_UNIT(LENGTH_MEASURE(0.001),#10266,
'DISTANCE_ACCURACY_VALUE',
'Maximum model space distance between geometric entities at asserted c
onnectivities');
#10240=(
GEOMETRIC_REPRESENTATION_CONTEXT(3)
GLOBAL_UNCERTAINTY_ASSIGNED_CONTEXT((#10202))
GLOBAL_UNIT_ASSIGNED_CONTEXT((#10266,#10268,#10269))
REPRESENTATION_CONTEXT('','3D')
);
#10265=(
GEOMETRIC_REPRESENTATION_CONTEXT(3)
GLOBAL_UNCERTAINTY_ASSIGNED_CONTEXT((#10227))
GLOBAL_UNIT_ASSIGNED_CONTEXT((#10266,#10268,#10269))
REPRESENTATION_CONTEXT('','3D')
);
#10266=(
LENGTH_UNIT()
NAMED_UNIT(*)
SI_UNIT(.CENTI.,.METRE.)
);
#10268=(
NAMED_UNIT(*)
PLANE_ANGLE_UNIT()
SI_UNIT($,.RADIAN.)
);
#10269=(
NAMED_UNIT(*)
SI_UNIT($,.STERADIAN.)
SOLID_ANGLE_UNIT()
);
#10282=SHAPE_DEFINITION_REPRESENTATION(#10319,#10416);
#10319=PRODUCT_DEFINITION_SHAPE('',$,#10454);
#10416=SHAPE_REPRESENTATION('',(#5647),#10240);
#10441=PRODUCT_DEFINITION_CONTEXT('part definition',#10554,'design');
#10454=PRODUCT_DEFINITION('Cylinder top cap','Cylinder top cap',#10491,
#10441);
#10491=PRODUCT_DEFINITION_FORMATION('',$,#10568);
#10554=APPLICATION_CONTEXT(
'Core Data for Automotive Mechanical Design Process');
#10555=PRODUCT_CONTEXT('part definition',#10554,'mechanical');
#10568=PRODUCT('Cylinder top cap','Cylinder top cap','Cylinder top cap',
(#10555));
#10642=COLOUR_RGB('Sky Blue',0.24,0.69,0.87);
#10643=FILL_AREA_STYLE_COLOUR('',#10642);
#10644=FILL_AREA_STYLE('',(#10643));
#10645=SURFACE_STYLE_FILL_AREA(#10644);
#10646=SURFACE_SIDE_STYLE('',(#10645));
#10647=SURFACE_STYLE_USAGE(.BOTH.,#10646);
#10648=PRESENTATION_STYLE_ASSIGNMENT((#10647));
ENDSEC;
END-ISO-10303-21;
